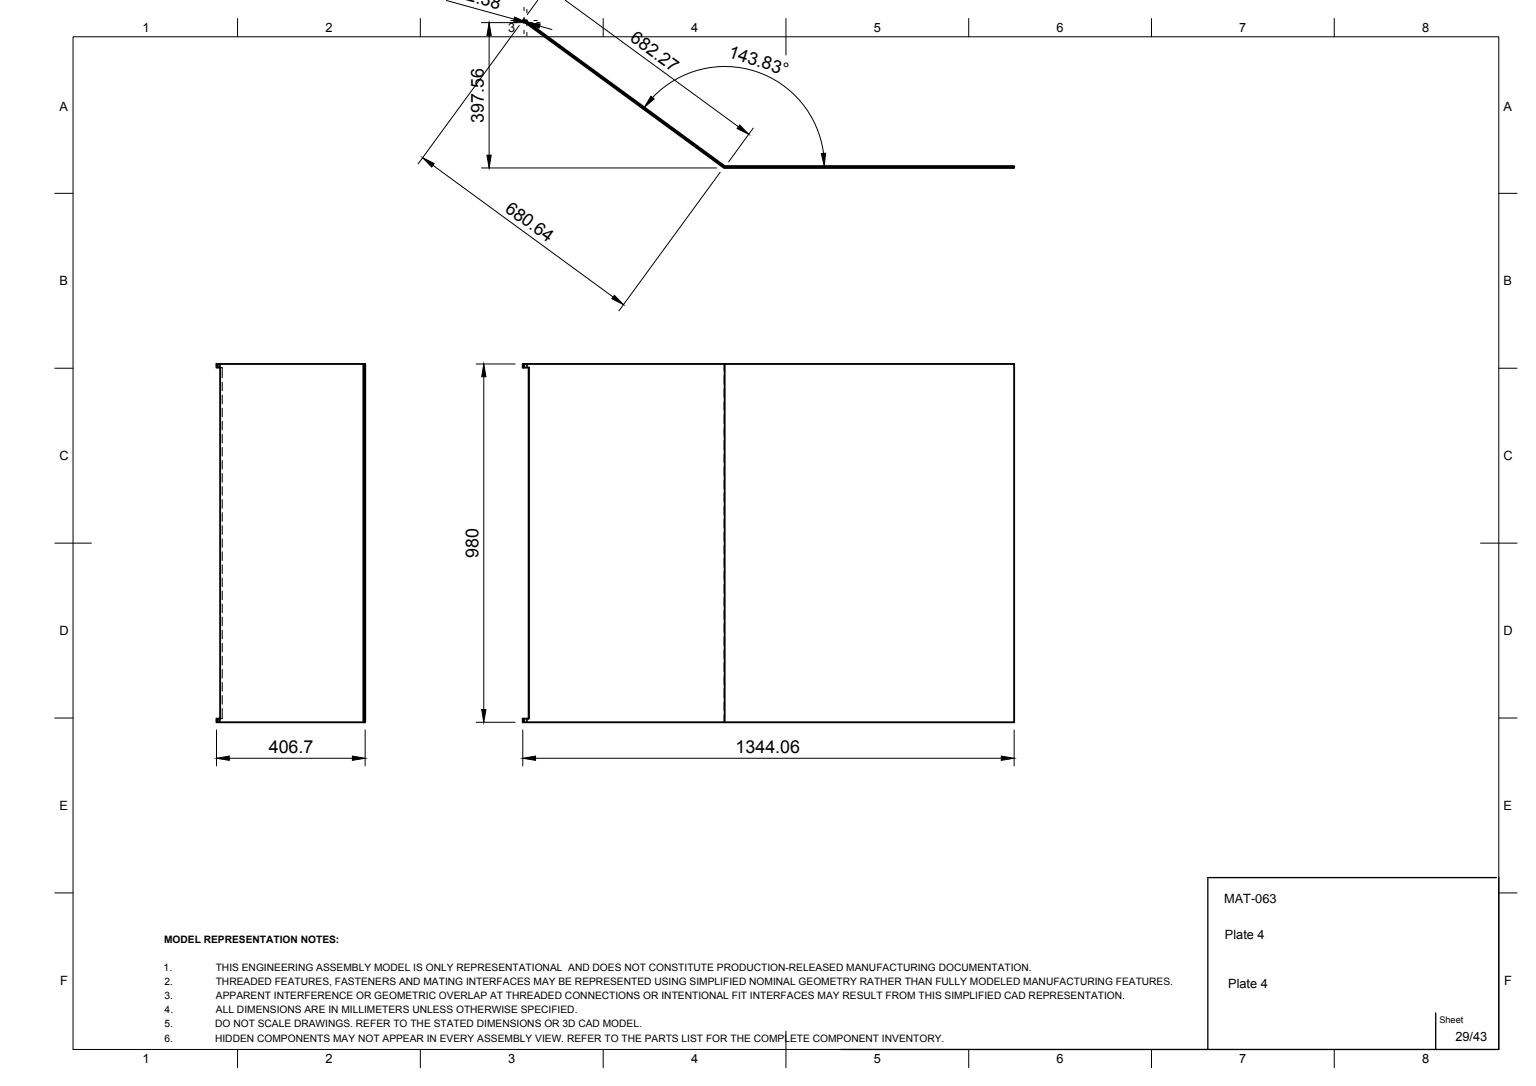
ISO-10303-21;
HEADER;
/* Generated by software containing ST-Developer
 * from STEP Tools, Inc. (www.steptools.com) 
 */

FILE_DESCRIPTION(
/* description */ (''),
/* implementation_level */ '2;1');

FILE_NAME(
/* name */ 'Plate 4.step',
/* time_stamp */ '2026-10-24T09:43:01-07:00',
/* author */ (''),
/* organization */ (''),
/* preprocessor_version */ 'ST-DEVELOPER v20.2',
/* originating_system */ 'Autodesk Translation Framework v15.15.0.0',
/* authorisation */ '');

FILE_SCHEMA (('AUTOMOTIVE_DESIGN { 1 0 10303 214 3 1 1 }'));
ENDSEC;

DATA;
#10=MECHANICAL_DESIGN_GEOMETRIC_PRESENTATION_REPRESENTATION('',(#294),#11112);
#228=SHAPE_REPRESENTATION_RELATIONSHIP('SRR','None',#11253,#261);
#261=ADVANCED_BREP_SHAPE_REPRESENTATION('',(#327),#11098);
#294=STYLED_ITEM('',(#11426),#327);
#327=MANIFOLD_SOLID_BREP('Plate 4',#6031);
#463=FACE_BOUND('',#1455,.T.);
#464=FACE_BOUND('',#1456,.T.);
#465=FACE_BOUND('',#1463,.T.);
#466=FACE_BOUND('',#1464,.T.);
#467=FACE_BOUND('',#1467,.T.);
#468=FACE_BOUND('',#1468,.T.);
#469=FACE_BOUND('',#1471,.T.);
#470=FACE_BOUND('',#1472,.T.);
#626=PLANE('',#7086);
#627=PLANE('',#7089);
#628=PLANE('',#7090);
#629=PLANE('',#7091);
#630=PLANE('',#7092);
#631=PLANE('',#7093);
#632=PLANE('',#7094);
#633=PLANE('',#7096);
#634=PLANE('',#7097);
#635=PLANE('',#7099);
#636=PLANE('',#7100);
#637=PLANE('',#7103);
#965=FACE_OUTER_BOUND('',#1453,.T.);
#966=FACE_OUTER_BOUND('',#1454,.T.);
#967=FACE_OUTER_BOUND('',#1457,.T.);
#968=FACE_OUTER_BOUND('',#1458,.T.);
#969=FACE_OUTER_BOUND('',#1459,.T.);
#970=FACE_OUTER_BOUND('',#1460,.T.);
#971=FACE_OUTER_BOUND('',#1461,.T.);
#972=FACE_OUTER_BOUND('',#1462,.T.);
#973=FACE_OUTER_BOUND('',#1465,.T.);
#974=FACE_OUTER_BOUND('',#1466,.T.);
#975=FACE_OUTER_BOUND('',#1469,.T.);
#976=FACE_OUTER_BOUND('',#1470,.T.);
#977=FACE_OUTER_BOUND('',#1473,.T.);
#978=FACE_OUTER_BOUND('',#1474,.T.);
#979=FACE_OUTER_BOUND('',#1475,.T.);
#980=FACE_OUTER_BOUND('',#1476,.T.);
#1453=EDGE_LOOP('',(#5209,#5210,#5211,#5212));
#1454=EDGE_LOOP('',(#5213,#5214,#5215,#5216,#5217,#5218));
#1455=EDGE_LOOP('',(#5219));
#1456=EDGE_LOOP('',(#5220));
#1457=EDGE_LOOP('',(#5221,#5222,#5223,#5224,#5225,#5226,#5227,#5228));
#1458=EDGE_LOOP('',(#5229,#5230,#5231,#5232));
#1459=EDGE_LOOP('',(#5233,#5234,#5235,#5236));
#1460=EDGE_LOOP('',(#5237,#5238,#5239,#5240));
#1461=EDGE_LOOP('',(#5241,#5242,#5243,#5244,#5245,#5246,#5247,#5248));
#1462=EDGE_LOOP('',(#5249,#5250,#5251,#5252));
#1463=EDGE_LOOP('',(#5253));
#1464=EDGE_LOOP('',(#5254));
#1465=EDGE_LOOP('',(#5255,#5256,#5257,#5258));
#1466=EDGE_LOOP('',(#5259,#5260,#5261,#5262,#5263,#5264));
#1467=EDGE_LOOP('',(#5265));
#1468=EDGE_LOOP('',(#5266));
#1469=EDGE_LOOP('',(#5267,#5268,#5269,#5270));
#1470=EDGE_LOOP('',(#5271,#5272,#5273,#5274));
#1471=EDGE_LOOP('',(#5275));
#1472=EDGE_LOOP('',(#5276));
#1473=EDGE_LOOP('',(#5277,#5278,#5279,#5280));
#1474=EDGE_LOOP('',(#5281,#5282,#5283,#5284));
#1475=EDGE_LOOP('',(#5285,#5286,#5287,#5288));
#1476=EDGE_LOOP('',(#5289,#5290,#5291,#5292));
#1834=LINE('',#10681,#2193);
#1835=LINE('',#10686,#2194);
#1836=LINE('',#10688,#2195);
#1837=LINE('',#10690,#2196);
#1838=LINE('',#10692,#2197);
#1839=LINE('',#10694,#2198);
#1840=LINE('',#10695,#2199);
#1841=LINE('',#10703,#2200);
#1842=LINE('',#10705,#2201);
#1843=LINE('',#10707,#2202);
#1844=LINE('',#10709,#2203);
#1845=LINE('',#10710,#2204);
#1846=LINE('',#10712,#2205);
#1847=LINE('',#10713,#2206);
#1848=LINE('',#10716,#2207);
#1849=LINE('',#10717,#2208);
#1850=LINE('',#10720,#2209);
#1851=LINE('',#10721,#2210);
#1852=LINE('',#10724,#2211);
#1853=LINE('',#10725,#2212);
#1854=LINE('',#10729,#2213);
#1855=LINE('',#10731,#2214);
#1856=LINE('',#10733,#2215);
#1857=LINE('',#10735,#2216);
#1858=LINE('',#10736,#2217);
#1859=LINE('',#10737,#2218);
#1860=LINE('',#10739,#2219);
#1861=LINE('',#10740,#2220);
#1862=LINE('',#10744,#2221);
#1863=LINE('',#10749,#2222);
#1864=LINE('',#10751,#2223);
#1865=LINE('',#10758,#2224);
#1866=LINE('',#10760,#2225);
#1867=LINE('',#10762,#2226);
#2193=VECTOR('',#8892,0.00118970099999992);
#2194=VECTOR('',#8897,0.01);
#2195=VECTOR('',#8898,0.01);
#2196=VECTOR('',#8899,0.01);
#2197=VECTOR('',#8900,0.01);
#2198=VECTOR('',#8901,0.01);
#2199=VECTOR('',#8902,0.01);
#2200=VECTOR('',#8909,0.01);
#2201=VECTOR('',#8910,0.01);
#2202=VECTOR('',#8911,0.01);
#2203=VECTOR('',#8912,0.01);
#2204=VECTOR('',#8913,0.01);
#2205=VECTOR('',#8914,0.01);
#2206=VECTOR('',#8915,0.01);
#2207=VECTOR('',#8918,0.01);
#2208=VECTOR('',#8919,0.01);
#2209=VECTOR('',#8922,0.01);
#2210=VECTOR('',#8923,0.01);
#2211=VECTOR('',#8926,0.01);
#2212=VECTOR('',#8927,0.01);
#2213=VECTOR('',#8930,0.01);
#2214=VECTOR('',#8931,0.01);
#2215=VECTOR('',#8932,0.01);
#2216=VECTOR('',#8933,0.01);
#2217=VECTOR('',#8934,0.01);
#2218=VECTOR('',#8935,0.01);
#2219=VECTOR('',#8938,0.01);
#2220=VECTOR('',#8939,0.01);
#2221=VECTOR('',#8944,0.01);
#2222=VECTOR('',#8951,0.01);
#2223=VECTOR('',#8954,0.01);
#2224=VECTOR('',#8963,0.00118970100010167);
#2225=VECTOR('',#8966,0.00118970100010167);
#2226=VECTOR('',#8969,0.00118970099999992);
#2628=CIRCLE('',#7084,0.00118970099999992);
#2629=CIRCLE('',#7085,0.00118970099999992);
#2630=CIRCLE('',#7087,0.00118970100010167);
#2631=CIRCLE('',#7088,0.00118970100010167);
#2632=CIRCLE('',#7095,0.00118970099999992);
#2633=CIRCLE('',#7098,0.00118970099999992);
#2634=CIRCLE('',#7101,0.00118970100010167);
#2635=CIRCLE('',#7102,0.00118970100010167);
#3082=VERTEX_POINT('',#10678);
#3083=VERTEX_POINT('',#10680);
#3084=VERTEX_POINT('',#10684);
#3085=VERTEX_POINT('',#10685);
#3086=VERTEX_POINT('',#10687);
#3087=VERTEX_POINT('',#10689);
#3088=VERTEX_POINT('',#10691);
#3089=VERTEX_POINT('',#10693);
#3090=VERTEX_POINT('',#10696);
#3091=VERTEX_POINT('',#10698);
#3092=VERTEX_POINT('',#10701);
#3093=VERTEX_POINT('',#10702);
#3094=VERTEX_POINT('',#10704);
#3095=VERTEX_POINT('',#10706);
#3096=VERTEX_POINT('',#10708);
#3097=VERTEX_POINT('',#10711);
#3098=VERTEX_POINT('',#10715);
#3099=VERTEX_POINT('',#10719);
#3100=VERTEX_POINT('',#10723);
#3101=VERTEX_POINT('',#10727);
#3102=VERTEX_POINT('',#10728);
#3103=VERTEX_POINT('',#10730);
#3104=VERTEX_POINT('',#10732);
#3105=VERTEX_POINT('',#10734);
#3106=VERTEX_POINT('',#10741);
#3107=VERTEX_POINT('',#10746);
#3108=VERTEX_POINT('',#10752);
#3109=VERTEX_POINT('',#10754);
#3808=EDGE_CURVE('',#3082,#3082,#2628,.T.);
#3809=EDGE_CURVE('',#3082,#3083,#1834,.T.);
#3810=EDGE_CURVE('',#3083,#3083,#2629,.F.);
#3811=EDGE_CURVE('',#3084,#3085,#1835,.T.);
#3812=EDGE_CURVE('',#3086,#3084,#1836,.T.);
#3813=EDGE_CURVE('',#3087,#3086,#1837,.T.);
#3814=EDGE_CURVE('',#3088,#3087,#1838,.T.);
#3815=EDGE_CURVE('',#3089,#3088,#1839,.T.);
#3816=EDGE_CURVE('',#3085,#3089,#1840,.T.);
#3817=EDGE_CURVE('',#3090,#3090,#2630,.T.);
#3818=EDGE_CURVE('',#3091,#3091,#2631,.T.);
#3819=EDGE_CURVE('',#3092,#3093,#1841,.T.);
#3820=EDGE_CURVE('',#3094,#3092,#1842,.T.);
#3821=EDGE_CURVE('',#3095,#3094,#1843,.T.);
#3822=EDGE_CURVE('',#3096,#3095,#1844,.T.);
#3823=EDGE_CURVE('',#3086,#3096,#1845,.T.);
#3824=EDGE_CURVE('',#3097,#3084,#1846,.T.);
#3825=EDGE_CURVE('',#3093,#3097,#1847,.T.);
#3826=EDGE_CURVE('',#3098,#3096,#1848,.T.);
#3827=EDGE_CURVE('',#3087,#3098,#1849,.T.);
#3828=EDGE_CURVE('',#3099,#3098,#1850,.T.);
#3829=EDGE_CURVE('',#3088,#3099,#1851,.T.);
#3830=EDGE_CURVE('',#3100,#3099,#1852,.T.);
#3831=EDGE_CURVE('',#3089,#3100,#1853,.T.);
#3832=EDGE_CURVE('',#3101,#3102,#1854,.T.);
#3833=EDGE_CURVE('',#3103,#3101,#1855,.T.);
#3834=EDGE_CURVE('',#3104,#3103,#1856,.T.);
#3835=EDGE_CURVE('',#3105,#3104,#1857,.T.);
#3836=EDGE_CURVE('',#3085,#3105,#1858,.T.);
#3837=EDGE_CURVE('',#3102,#3100,#1859,.T.);
#3838=EDGE_CURVE('',#3101,#3094,#1860,.T.);
#3839=EDGE_CURVE('',#3092,#3103,#1861,.T.);
#3840=EDGE_CURVE('',#3106,#3106,#2632,.F.);
#3841=EDGE_CURVE('',#3095,#3102,#1862,.T.);
#3842=EDGE_CURVE('',#3107,#3107,#2633,.T.);
#3843=EDGE_CURVE('',#3097,#3105,#1863,.T.);
#3844=EDGE_CURVE('',#3093,#3104,#1864,.T.);
#3845=EDGE_CURVE('',#3108,#3108,#2634,.F.);
#3846=EDGE_CURVE('',#3109,#3109,#2635,.F.);
#3847=EDGE_CURVE('',#3109,#3091,#1865,.T.);
#3848=EDGE_CURVE('',#3108,#3090,#1866,.T.);
#3849=EDGE_CURVE('',#3107,#3106,#1867,.T.);
#5209=ORIENTED_EDGE('',*,*,#3808,.F.);
#5210=ORIENTED_EDGE('',*,*,#3809,.T.);
#5211=ORIENTED_EDGE('',*,*,#3810,.F.);
#5212=ORIENTED_EDGE('',*,*,#3809,.F.);
#5213=ORIENTED_EDGE('',*,*,#3811,.F.);
#5214=ORIENTED_EDGE('',*,*,#3812,.F.);
#5215=ORIENTED_EDGE('',*,*,#3813,.F.);
#5216=ORIENTED_EDGE('',*,*,#3814,.F.);
#5217=ORIENTED_EDGE('',*,*,#3815,.F.);
#5218=ORIENTED_EDGE('',*,*,#3816,.F.);
#5219=ORIENTED_EDGE('',*,*,#3817,.F.);
#5220=ORIENTED_EDGE('',*,*,#3818,.F.);
#5221=ORIENTED_EDGE('',*,*,#3819,.F.);
#5222=ORIENTED_EDGE('',*,*,#3820,.F.);
#5223=ORIENTED_EDGE('',*,*,#3821,.F.);
#5224=ORIENTED_EDGE('',*,*,#3822,.F.);
#5225=ORIENTED_EDGE('',*,*,#3823,.F.);
#5226=ORIENTED_EDGE('',*,*,#3812,.T.);
#5227=ORIENTED_EDGE('',*,*,#3824,.F.);
#5228=ORIENTED_EDGE('',*,*,#3825,.F.);
#5229=ORIENTED_EDGE('',*,*,#3826,.F.);
#5230=ORIENTED_EDGE('',*,*,#3827,.F.);
#5231=ORIENTED_EDGE('',*,*,#3813,.T.);
#5232=ORIENTED_EDGE('',*,*,#3823,.T.);
#5233=ORIENTED_EDGE('',*,*,#3828,.F.);
#5234=ORIENTED_EDGE('',*,*,#3829,.F.);
#5235=ORIENTED_EDGE('',*,*,#3814,.T.);
#5236=ORIENTED_EDGE('',*,*,#3827,.T.);
#5237=ORIENTED_EDGE('',*,*,#3830,.F.);
#5238=ORIENTED_EDGE('',*,*,#3831,.F.);
#5239=ORIENTED_EDGE('',*,*,#3815,.T.);
#5240=ORIENTED_EDGE('',*,*,#3829,.T.);
#5241=ORIENTED_EDGE('',*,*,#3832,.F.);
#5242=ORIENTED_EDGE('',*,*,#3833,.F.);
#5243=ORIENTED_EDGE('',*,*,#3834,.F.);
#5244=ORIENTED_EDGE('',*,*,#3835,.F.);
#5245=ORIENTED_EDGE('',*,*,#3836,.F.);
#5246=ORIENTED_EDGE('',*,*,#3816,.T.);
#5247=ORIENTED_EDGE('',*,*,#3831,.T.);
#5248=ORIENTED_EDGE('',*,*,#3837,.F.);
#5249=ORIENTED_EDGE('',*,*,#3833,.T.);
#5250=ORIENTED_EDGE('',*,*,#3838,.T.);
#5251=ORIENTED_EDGE('',*,*,#3820,.T.);
#5252=ORIENTED_EDGE('',*,*,#3839,.T.);
#5253=ORIENTED_EDGE('',*,*,#3840,.T.);
#5254=ORIENTED_EDGE('',*,*,#3810,.T.);
#5255=ORIENTED_EDGE('',*,*,#3821,.T.);
#5256=ORIENTED_EDGE('',*,*,#3838,.F.);
#5257=ORIENTED_EDGE('',*,*,#3832,.T.);
#5258=ORIENTED_EDGE('',*,*,#3841,.F.);
#5259=ORIENTED_EDGE('',*,*,#3841,.T.);
#5260=ORIENTED_EDGE('',*,*,#3837,.T.);
#5261=ORIENTED_EDGE('',*,*,#3830,.T.);
#5262=ORIENTED_EDGE('',*,*,#3828,.T.);
#5263=ORIENTED_EDGE('',*,*,#3826,.T.);
#5264=ORIENTED_EDGE('',*,*,#3822,.T.);
#5265=ORIENTED_EDGE('',*,*,#3842,.T.);
#5266=ORIENTED_EDGE('',*,*,#3808,.T.);
#5267=ORIENTED_EDGE('',*,*,#3811,.T.);
#5268=ORIENTED_EDGE('',*,*,#3836,.T.);
#5269=ORIENTED_EDGE('',*,*,#3843,.F.);
#5270=ORIENTED_EDGE('',*,*,#3824,.T.);
#5271=ORIENTED_EDGE('',*,*,#3835,.T.);
#5272=ORIENTED_EDGE('',*,*,#3844,.F.);
#5273=ORIENTED_EDGE('',*,*,#3825,.T.);
#5274=ORIENTED_EDGE('',*,*,#3843,.T.);
#5275=ORIENTED_EDGE('',*,*,#3845,.F.);
#5276=ORIENTED_EDGE('',*,*,#3846,.F.);
#5277=ORIENTED_EDGE('',*,*,#3834,.T.);
#5278=ORIENTED_EDGE('',*,*,#3839,.F.);
#5279=ORIENTED_EDGE('',*,*,#3819,.T.);
#5280=ORIENTED_EDGE('',*,*,#3844,.T.);
#5281=ORIENTED_EDGE('',*,*,#3846,.T.);
#5282=ORIENTED_EDGE('',*,*,#3847,.T.);
#5283=ORIENTED_EDGE('',*,*,#3818,.T.);
#5284=ORIENTED_EDGE('',*,*,#3847,.F.);
#5285=ORIENTED_EDGE('',*,*,#3845,.T.);
#5286=ORIENTED_EDGE('',*,*,#3848,.T.);
#5287=ORIENTED_EDGE('',*,*,#3817,.T.);
#5288=ORIENTED_EDGE('',*,*,#3848,.F.);
#5289=ORIENTED_EDGE('',*,*,#3842,.F.);
#5290=ORIENTED_EDGE('',*,*,#3849,.T.);
#5291=ORIENTED_EDGE('',*,*,#3840,.F.);
#5292=ORIENTED_EDGE('',*,*,#3849,.F.);
#5613=CYLINDRICAL_SURFACE('',#7083,0.00118970099999992);
#5614=CYLINDRICAL_SURFACE('',#7104,0.00118970100010167);
#5615=CYLINDRICAL_SURFACE('',#7105,0.00118970100010167);
#5616=CYLINDRICAL_SURFACE('',#7106,0.00118970099999992);
#5938=ADVANCED_FACE('',(#965),#5613,.F.);
#5939=ADVANCED_FACE('',(#966,#463,#464),#626,.F.);
#5940=ADVANCED_FACE('',(#967),#627,.F.);
#5941=ADVANCED_FACE('',(#968),#628,.F.);
#5942=ADVANCED_FACE('',(#969),#629,.F.);
#5943=ADVANCED_FACE('',(#970),#630,.F.);
#5944=ADVANCED_FACE('',(#971),#631,.F.);
#5945=ADVANCED_FACE('',(#972,#465,#466),#632,.T.);
#5946=ADVANCED_FACE('',(#973),#633,.F.);
#5947=ADVANCED_FACE('',(#974,#467,#468),#634,.T.);
#5948=ADVANCED_FACE('',(#975),#635,.F.);
#5949=ADVANCED_FACE('',(#976,#469,#470),#636,.F.);
#5950=ADVANCED_FACE('',(#977),#637,.F.);
#5951=ADVANCED_FACE('',(#978),#5614,.F.);
#5952=ADVANCED_FACE('',(#979),#5615,.F.);
#5953=ADVANCED_FACE('',(#980),#5616,.F.);
#6031=CLOSED_SHELL('',(#5938,#5939,#5940,#5941,#5942,#5943,#5944,#5945,
#5946,#5947,#5948,#5949,#5950,#5951,#5952,#5953));
#7082=AXIS2_PLACEMENT_3D('',#10676,#8886,#8887);
#7083=AXIS2_PLACEMENT_3D('',#10677,#8888,#8889);
#7084=AXIS2_PLACEMENT_3D('',#10679,#8890,#8891);
#7085=AXIS2_PLACEMENT_3D('',#10682,#8893,#8894);
#7086=AXIS2_PLACEMENT_3D('',#10683,#8895,#8896);
#7087=AXIS2_PLACEMENT_3D('',#10697,#8903,#8904);
#7088=AXIS2_PLACEMENT_3D('',#10699,#8905,#8906);
#7089=AXIS2_PLACEMENT_3D('',#10700,#8907,#8908);
#7090=AXIS2_PLACEMENT_3D('',#10714,#8916,#8917);
#7091=AXIS2_PLACEMENT_3D('',#10718,#8920,#8921);
#7092=AXIS2_PLACEMENT_3D('',#10722,#8924,#8925);
#7093=AXIS2_PLACEMENT_3D('',#10726,#8928,#8929);
#7094=AXIS2_PLACEMENT_3D('',#10738,#8936,#8937);
#7095=AXIS2_PLACEMENT_3D('',#10742,#8940,#8941);
#7096=AXIS2_PLACEMENT_3D('',#10743,#8942,#8943);
#7097=AXIS2_PLACEMENT_3D('',#10745,#8945,#8946);
#7098=AXIS2_PLACEMENT_3D('',#10747,#8947,#8948);
#7099=AXIS2_PLACEMENT_3D('',#10748,#8949,#8950);
#7100=AXIS2_PLACEMENT_3D('',#10750,#8952,#8953);
#7101=AXIS2_PLACEMENT_3D('',#10753,#8955,#8956);
#7102=AXIS2_PLACEMENT_3D('',#10755,#8957,#8958);
#7103=AXIS2_PLACEMENT_3D('',#10756,#8959,#8960);
#7104=AXIS2_PLACEMENT_3D('',#10757,#8961,#8962);
#7105=AXIS2_PLACEMENT_3D('',#10759,#8964,#8965);
#7106=AXIS2_PLACEMENT_3D('',#10761,#8967,#8968);
#8886=DIRECTION('axis',(0.,0.,1.));
#8887=DIRECTION('refdir',(1.,0.,0.));
#8888=DIRECTION('center_axis',(1.,0.,0.));
#8889=DIRECTION('ref_axis',(0.,0.,-1.));
#8890=DIRECTION('center_axis',(1.,0.,0.));
#8891=DIRECTION('ref_axis',(0.,0.,-1.));
#8892=DIRECTION('',(1.,0.,0.));
#8893=DIRECTION('center_axis',(1.,0.,0.));
#8894=DIRECTION('ref_axis',(0.,0.,-1.));
#8895=DIRECTION('center_axis',(-1.,-3.44325444684946E-17,-2.70173859336735E-18));
#8896=DIRECTION('ref_axis',(3.44325444684946E-17,-1.,-2.77218243538616E-51));
#8897=DIRECTION('',(0.,0.866025402838329,0.50000000163871));
#8898=DIRECTION('',(0.,-0.499999999594076,0.866025404018799));
#8899=DIRECTION('',(0.,0.107473447068807,0.994207955196069));
#8900=DIRECTION('',(0.,-0.994207960742926,0.107473395756311));
#8901=DIRECTION('',(0.,-0.107473446602436,-0.994207955246483));
#8902=DIRECTION('',(0.,0.499999999523326,-0.866025404059647));
#8903=DIRECTION('center_axis',(1.,0.,9.33194999941347E-14));
#8904=DIRECTION('ref_axis',(9.33194999941347E-14,0.,-1.));
#8905=DIRECTION('center_axis',(1.,0.,9.33194999941347E-14));
#8906=DIRECTION('ref_axis',(9.33194999941347E-14,0.,-1.));
#8907=DIRECTION('center_axis',(2.32889998828464E-18,0.866025404018799,0.499999999594076));
#8908=DIRECTION('ref_axis',(-1.13747398687096E-34,-0.499999999594076,0.866025404018799));
#8909=DIRECTION('',(1.,0.,0.));
#8910=DIRECTION('',(0.,0.499999999594074,-0.8660254040188));
#8911=DIRECTION('',(1.,0.,0.));
#8912=DIRECTION('',(0.,-0.499999999594075,0.866025404018799));
#8913=DIRECTION('',(-1.,0.,0.));
#8914=DIRECTION('',(1.,0.,0.));
#8915=DIRECTION('',(0.,-0.499999999594074,0.8660254040188));
#8916=DIRECTION('center_axis',(-2.99047289596199E-18,0.994207955196069,
-0.107473447068807));
#8917=DIRECTION('ref_axis',(1.7192384968967E-36,0.107473447068807,0.994207955196069));
#8918=DIRECTION('',(0.,0.107473447068808,0.994207955196069));
#8919=DIRECTION('',(-1.,0.,0.));
#8920=DIRECTION('center_axis',(-3.44011407178642E-19,0.10747339575632,0.994207960742925));
#8921=DIRECTION('ref_axis',(-9.20601768266839E-37,-0.994207960742925,0.10747339575632));
#8922=DIRECTION('',(0.,-0.994207960742924,0.107473395756334));
#8923=DIRECTION('',(-1.,0.,0.));
#8924=DIRECTION('center_axis',(1.21066295142474E-17,-0.994207955246483,
0.107473446602436));
#8925=DIRECTION('ref_axis',(-1.21784695446604E-33,-0.107473446602436,-0.994207955246483));
#8926=DIRECTION('',(0.,-0.107473446602435,-0.994207955246483));
#8927=DIRECTION('',(-1.,0.,0.));
#8928=DIRECTION('center_axis',(2.27934427627508E-17,-0.866025404059647,
-0.499999999523326));
#8929=DIRECTION('ref_axis',(9.40315152180257E-34,0.499999999523326,-0.866025404059647));
#8930=DIRECTION('',(-1.,0.,0.));
#8931=DIRECTION('',(0.,-0.499999999523324,0.866025404059648));
#8932=DIRECTION('',(-1.,0.,0.));
#8933=DIRECTION('',(0.,0.499999999523324,-0.866025404059648));
#8934=DIRECTION('',(-1.,0.,0.));
#8935=DIRECTION('',(0.,0.499999999523327,-0.866025404059646));
#8936=DIRECTION('center_axis',(1.,-3.36352380295954E-15,-3.1884171780454E-16));
#8937=DIRECTION('ref_axis',(3.36352380295954E-15,1.,-1.57533431125151E-47));
#8938=DIRECTION('',(0.,-0.866025402838331,-0.500000001638706));
#8939=DIRECTION('',(0.,1.,0.));
#8940=DIRECTION('center_axis',(1.,0.,0.));
#8941=DIRECTION('ref_axis',(0.,0.,-1.));
#8942=DIRECTION('center_axis',(1.86029643864781E-15,0.500000001638701,-0.866025402838334));
#8943=DIRECTION('ref_axis',(-2.70969563331381E-32,0.866025402838334,0.500000001638701));
#8944=DIRECTION('',(0.,0.866025402838314,0.500000001638735));
#8945=DIRECTION('center_axis',(-1.,3.44325444684946E-17,2.70173859336735E-18));
#8946=DIRECTION('ref_axis',(-3.44325444684946E-17,-1.,-2.77218243538616E-51));
#8947=DIRECTION('center_axis',(1.,0.,0.));
#8948=DIRECTION('ref_axis',(0.,0.,-1.));
#8949=DIRECTION('center_axis',(1.86511836885772E-15,0.500000001638701,-0.866025402838334));
#8950=DIRECTION('ref_axis',(-6.80058163600059E-32,0.866025402838334,0.500000001638701));
#8951=DIRECTION('',(0.,0.866025402838379,0.500000001638623));
#8952=DIRECTION('center_axis',(1.,3.36352380295954E-15,3.1884171780454E-16));
#8953=DIRECTION('ref_axis',(-3.36352380295954E-15,1.,-1.57533431125151E-47));
#8954=DIRECTION('',(0.,1.,0.));
#8955=DIRECTION('center_axis',(1.,0.,9.33194999941347E-14));
#8956=DIRECTION('ref_axis',(9.33194999941347E-14,0.,-1.));
#8957=DIRECTION('center_axis',(1.,0.,9.33194999941347E-14));
#8958=DIRECTION('ref_axis',(9.33194999941347E-14,0.,-1.));
#8959=DIRECTION('center_axis',(-1.82558994376595E-17,5.45297246983656E-15,
-1.));
#8960=DIRECTION('ref_axis',(0.,1.,5.45297246983656E-15));
#8961=DIRECTION('center_axis',(1.,0.,9.33194999941347E-14));
#8962=DIRECTION('ref_axis',(9.33194999941347E-14,0.,-1.));
#8963=DIRECTION('',(1.,0.,9.33194999941347E-14));
#8964=DIRECTION('center_axis',(1.,0.,9.33194999941347E-14));
#8965=DIRECTION('ref_axis',(9.33194999941347E-14,0.,-1.));
#8966=DIRECTION('',(1.,0.,9.33194999941347E-14));
#8967=DIRECTION('center_axis',(1.,0.,0.));
#8968=DIRECTION('ref_axis',(0.,0.,-1.));
#8969=DIRECTION('',(1.,0.,0.));
#10676=CARTESIAN_POINT('',(0.,0.,0.));
#10677=CARTESIAN_POINT('Origin',(-0.61,-0.537960337,0.967343188));
#10678=CARTESIAN_POINT('',(-0.49,-0.537960337,0.968532889));
#10679=CARTESIAN_POINT('Origin',(-0.49,-0.537960337,0.967343188));
#10680=CARTESIAN_POINT('',(-0.48,-0.537960337,0.968532889));
#10681=CARTESIAN_POINT('',(-0.61,-0.537960337,0.968532889));
#10682=CARTESIAN_POINT('Origin',(-0.48,-0.537960337,0.967343188));
#10683=CARTESIAN_POINT('Origin',(0.49,-0.3734279375,0.289236489));
#10684=CARTESIAN_POINT('',(0.489999999999839,-0.546160549999463,0.97651034600006));
#10685=CARTESIAN_POINT('',(0.489999999999929,-0.541830422999722,0.979010345999397));
#10686=CARTESIAN_POINT('',(0.49,-0.546160549333911,0.976510346384566));
#10687=CARTESIAN_POINT('',(0.49,-0.205841846999809,0.387061060999092));
#10688=CARTESIAN_POINT('',(0.49,-0.205841846899785,0.387061060826422));
#10689=CARTESIAN_POINT('',(0.489999999999528,-0.290922804999604,-0.400000000000061));
#10690=CARTESIAN_POINT('',(0.49,-0.290922805000769,-0.400000000007112));
#10691=CARTESIAN_POINT('',(0.489999999999528,-0.285951764999811,-0.400537366999761));
#10692=CARTESIAN_POINT('',(0.49,-0.28595176493698,-0.400537367006812));
#10693=CARTESIAN_POINT('',(0.49,-0.200695325999748,0.388147024998802));
#10694=CARTESIAN_POINT('',(0.49,-0.20069532607737,0.388147024284284));
#10695=CARTESIAN_POINT('',(0.49,-0.541830422462856,0.979010345069641));
#10696=CARTESIAN_POINT('',(0.49,-0.542782557,0.976885219000204));
#10697=CARTESIAN_POINT('Origin',(0.49,-0.542782557,0.975695518000103));
#10698=CARTESIAN_POINT('',(0.49,-0.537960337,0.968532889000204));
#10699=CARTESIAN_POINT('Origin',(0.49,-0.537960337,0.967343188000103));
#10700=CARTESIAN_POINT('Origin',(-5.27355936696949E-17,-0.3760011985,0.6817857035));
#10701=CARTESIAN_POINT('',(-0.479999999999998,-0.537552110829253,0.961600091996557));
#10702=CARTESIAN_POINT('',(0.479999999999998,-0.537552110829253,0.961600091996557));
#10703=CARTESIAN_POINT('',(-0.479999999395,-0.537552110814951,0.961600092000007));
#10704=CARTESIAN_POINT('',(-0.479999999999894,-0.546160550000244,0.976510345999441));
#10705=CARTESIAN_POINT('',(-0.48,-0.54616054991492,0.976510345852638));
#10706=CARTESIAN_POINT('',(-0.489999999999894,-0.546160549999321,0.976510346000143));
#10707=CARTESIAN_POINT('',(-0.489999999755,-0.54616055,0.976510346));
#10708=CARTESIAN_POINT('',(-0.49,-0.205841846999808,0.387061060999092));
#10709=CARTESIAN_POINT('',(-0.49,-0.20584184708508,0.387061061147362));
#10710=CARTESIAN_POINT('',(0.489999999755,-0.205841847,0.387061061));
#10711=CARTESIAN_POINT('',(0.479999999999928,-0.546160550000382,0.976510345999348));
#10712=CARTESIAN_POINT('',(0.479999999971875,-0.54616055,0.976510346));
#10713=CARTESIAN_POINT('',(0.48,-0.537552110906866,0.961600092100691));
#10714=CARTESIAN_POINT('Origin',(-5.27355936696949E-17,-0.248382326,-0.00646946950000008));
#10715=CARTESIAN_POINT('',(-0.48999999999979,-0.290922804999483,-0.400000000000166));
#10716=CARTESIAN_POINT('',(-0.49,-0.29092280497873,-0.399999999803235));
#10717=CARTESIAN_POINT('',(0.489999999755,-0.290922805,-0.4));
#10718=CARTESIAN_POINT('Origin',(-5.27355936696949E-17,-0.288437285,-0.4002686835));
#10719=CARTESIAN_POINT('',(-0.489999999999528,-0.285951764999492,-0.400537366999852));
#10720=CARTESIAN_POINT('',(-0.49,-0.285951765001243,-0.400537366999866));
#10721=CARTESIAN_POINT('',(0.489999999755,-0.285951765,-0.400537367));
#10722=CARTESIAN_POINT('Origin',(-5.27355936696949E-17,-0.243323545500001,
-0.00619517099999993));
#10723=CARTESIAN_POINT('',(-0.49,-0.200695325999748,0.388147024998802));
#10724=CARTESIAN_POINT('',(-0.49,-0.200695326026299,0.388147024756719));
#10725=CARTESIAN_POINT('',(0.489999999755,-0.200695326000001,0.388147025));
#10726=CARTESIAN_POINT('Origin',(-5.27355936696949E-17,-0.3712628745,0.6835786855));
#10727=CARTESIAN_POINT('',(-0.479999999999952,-0.541830423000291,0.979010345999481));
#10728=CARTESIAN_POINT('',(-0.489999999999929,-0.541830422999722,0.979010345999397));
#10729=CARTESIAN_POINT('',(-0.479999999971875,-0.541830423,0.979010346000001));
#10730=CARTESIAN_POINT('',(-0.479999999999922,-0.531778608197404,0.961600092003128));
#10731=CARTESIAN_POINT('',(-0.48,-0.531778608296587,0.961600092203291));
#10732=CARTESIAN_POINT('',(0.479999999999995,-0.531778608197352,0.961600092003097));
#10733=CARTESIAN_POINT('',(0.479999999395,-0.531778608211303,0.961600092000007));
#10734=CARTESIAN_POINT('',(0.479999999999952,-0.541830423000291,0.979010345999482));
#10735=CARTESIAN_POINT('',(0.48,-0.541830422911468,0.979010345846659));
#10736=CARTESIAN_POINT('',(0.489999999755,-0.541830423,0.979010346000001));
#10737=CARTESIAN_POINT('',(-0.49,-0.541830422710406,0.979010345498409));
#10738=CARTESIAN_POINT('Origin',(-0.48,-0.5389695795,0.970305218737048));
#10739=CARTESIAN_POINT('',(-0.48,-0.541830423513964,0.979010345703262));
#10740=CARTESIAN_POINT('',(-0.48,-0.537552111040899,0.961600092));
#10741=CARTESIAN_POINT('',(-0.48,-0.542782557,0.976885219));
#10742=CARTESIAN_POINT('Origin',(-0.48,-0.542782557,0.975695518));
#10743=CARTESIAN_POINT('Origin',(-0.485,-0.543995486499999,0.977760346));
#10744=CARTESIAN_POINT('',(-0.49,-0.546160549666815,0.976510346192364));
#10745=CARTESIAN_POINT('Origin',(-0.49,-0.3734279375,0.289236489));
#10746=CARTESIAN_POINT('',(-0.49,-0.542782557,0.976885219));
#10747=CARTESIAN_POINT('Origin',(-0.49,-0.542782557,0.975695518));
#10748=CARTESIAN_POINT('Origin',(0.485,-0.543995486499999,0.977760346));
#10749=CARTESIAN_POINT('',(0.48,-0.54616055,0.976510346));
#10750=CARTESIAN_POINT('Origin',(0.48,-0.5389695795,0.970305218737048));
#10751=CARTESIAN_POINT('',(0.48,-0.537552111040899,0.961600092));
#10752=CARTESIAN_POINT('',(0.48,-0.542782557,0.976885219000204));
#10753=CARTESIAN_POINT('Origin',(0.48,-0.542782557,0.975695518000102));
#10754=CARTESIAN_POINT('',(0.48,-0.537960337,0.968532889000204));
#10755=CARTESIAN_POINT('Origin',(0.48,-0.537960337,0.967343188000102));
#10756=CARTESIAN_POINT('Origin',(8.79851747015437E-17,-0.5346653595,0.961600092000007));
#10757=CARTESIAN_POINT('Origin',(-0.61,-0.537960337,0.967343188));
#10758=CARTESIAN_POINT('',(-0.61,-0.537960337,0.968532889000102));
#10759=CARTESIAN_POINT('Origin',(-0.61,-0.542782557,0.975695518));
#10760=CARTESIAN_POINT('',(-0.61,-0.542782557,0.976885219000102));
#10761=CARTESIAN_POINT('Origin',(-0.61,-0.542782557,0.975695518));
#10762=CARTESIAN_POINT('',(-0.61,-0.542782557,0.976885219));
#11059=UNCERTAINTY_MEASURE_WITH_UNIT(LENGTH_MEASURE(1.E-5),#11113,
'DISTANCE_ACCURACY_VALUE',
'Maximum model space distance between geometric entities at asserted c
onnectivities');
#11073=UNCERTAINTY_MEASURE_WITH_UNIT(LENGTH_MEASURE(1.E-5),#11113,
'DISTANCE_ACCURACY_VALUE',
'Maximum model space distance between geometric entities at asserted c
onnectivities');
#11098=(
GEOMETRIC_REPRESENTATION_CONTEXT(3)
GLOBAL_UNCERTAINTY_ASSIGNED_CONTEXT((#11059))
GLOBAL_UNIT_ASSIGNED_CONTEXT((#11113,#11114,#11115))
REPRESENTATION_CONTEXT('','3D')
);
#11112=(
GEOMETRIC_REPRESENTATION_CONTEXT(3)
GLOBAL_UNCERTAINTY_ASSIGNED_CONTEXT((#11073))
GLOBAL_UNIT_ASSIGNED_CONTEXT((#11113,#11114,#11115))
REPRESENTATION_CONTEXT('','3D')
);
#11113=(
LENGTH_UNIT()
NAMED_UNIT(*)
SI_UNIT($,.METRE.)
);
#11114=(
NAMED_UNIT(*)
PLANE_ANGLE_UNIT()
SI_UNIT($,.RADIAN.)
);
#11115=(
NAMED_UNIT(*)
SI_UNIT($,.STERADIAN.)
SOLID_ANGLE_UNIT()
);
#11140=SHAPE_DEFINITION_REPRESENTATION(#11185,#11253);
#11185=PRODUCT_DEFINITION_SHAPE('',$,#11292);
#11253=SHAPE_REPRESENTATION('',(#7082),#11098);
#11267=PRODUCT_DEFINITION_CONTEXT('part definition',#11383,'design');
#11292=PRODUCT_DEFINITION('Plate 4','Plate 4',#11330,#11267);
#11330=PRODUCT_DEFINITION_FORMATION('',$,#11409);
#11383=APPLICATION_CONTEXT(
'Core Data for Automotive Mechanical Design Process');
#11384=PRODUCT_CONTEXT('part definition',#11383,'mechanical');
#11409=PRODUCT('Plate 4','Plate 4','all_plates__ DE       35',(#11384));
#11426=PRESENTATION_STYLE_ASSIGNMENT((#11430));
#11430=SURFACE_STYLE_USAGE(.BOTH.,#11434);
#11434=SURFACE_SIDE_STYLE('',(#11438));
#11438=SURFACE_STYLE_FILL_AREA(#11442);
#11442=FILL_AREA_STYLE('Opaque(202,209,238)',(#11446));
#11446=FILL_AREA_STYLE_COLOUR('Opaque(202,209,238)',#11450);
#11450=COLOUR_RGB('Opaque(202,209,238)',0.792156862745098,0.819607843137255,
0.933333333333333);
ENDSEC;
END-ISO-10303-21;
